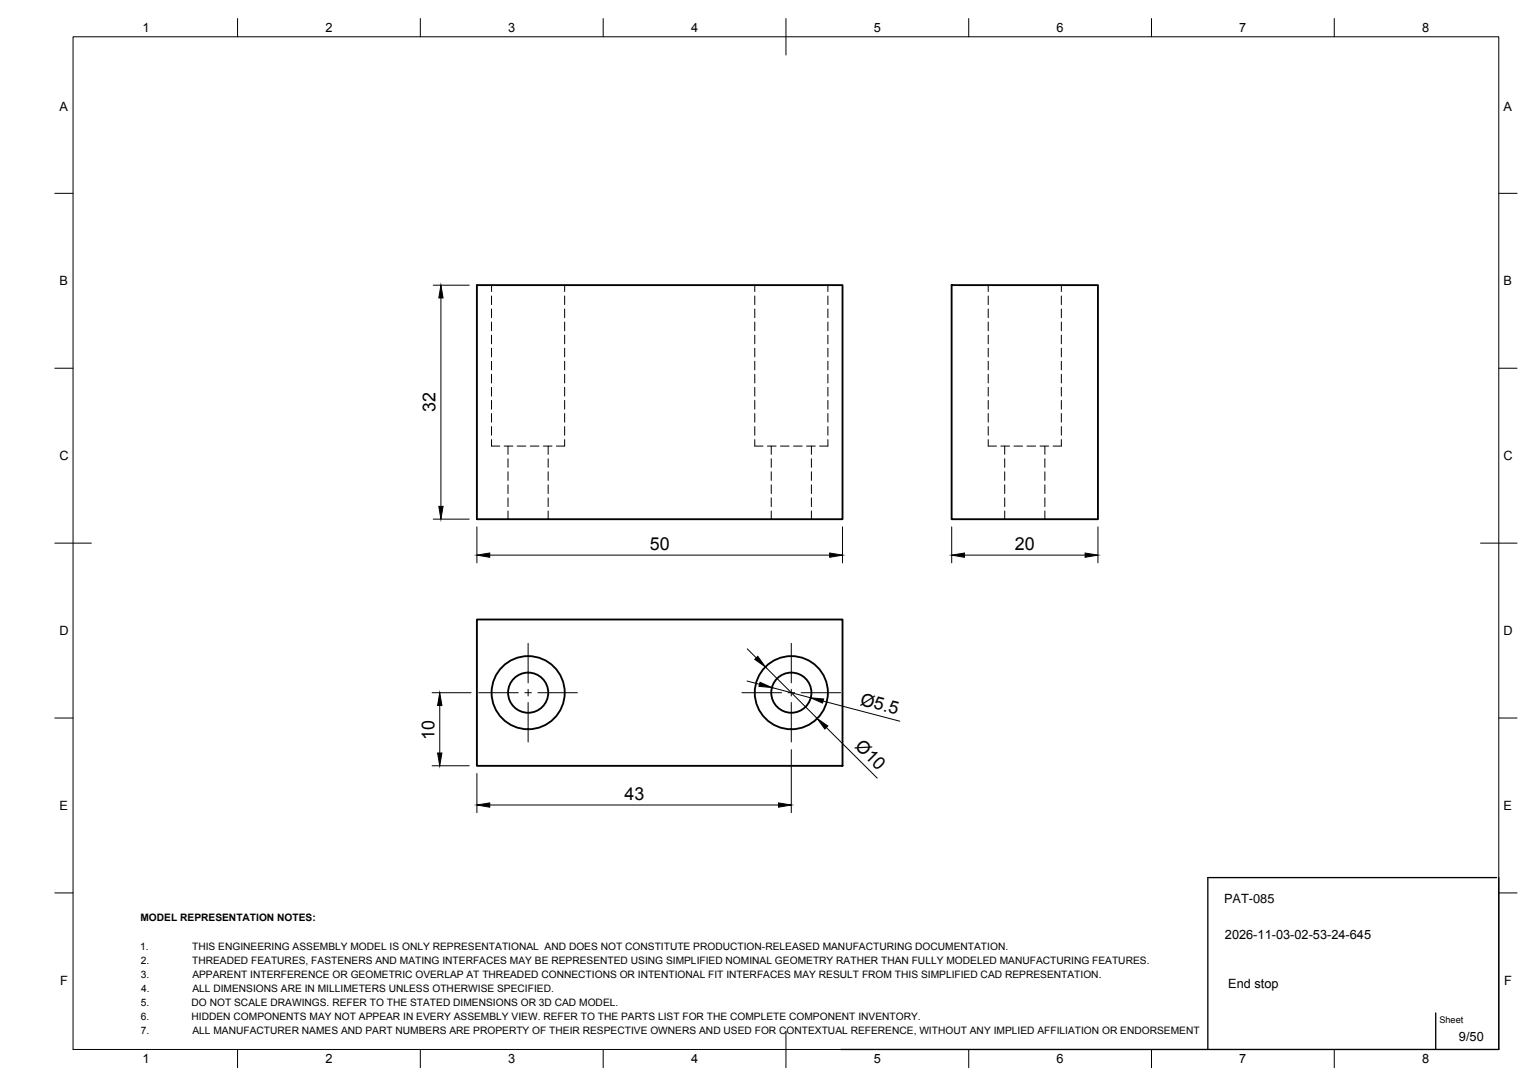
ISO-10303-21;
HEADER;
/* Generated by software containing ST-Developer
 * from STEP Tools, Inc. (www.steptools.com) 
 */

FILE_DESCRIPTION(
/* description */ ('Rack and pinion manual slide'),
/* implementation_level */ '2;1');

FILE_NAME(
/* name */ 'End stop.step',
/* time_stamp */ '2026-10-28T03:22:49-07:00',
/* author */ (''),
/* organization */ (''),
/* preprocessor_version */ 'ST-DEVELOPER v20.2',
/* originating_system */ 'Autodesk Translation Framework v15.17.0.0',
/* authorisation */ '');

FILE_SCHEMA (('AUTOMOTIVE_DESIGN { 1 0 10303 214 3 1 1 }'));
ENDSEC;

DATA;
#10=MECHANICAL_DESIGN_GEOMETRIC_PRESENTATION_REPRESENTATION('',(#736),#34851);
#644=SHAPE_REPRESENTATION_RELATIONSHIP('SRR','None',#35079,#690);
#690=ADVANCED_BREP_SHAPE_REPRESENTATION('',(#789),#34804);
#736=STYLED_ITEM('',(#35404),#789);
#789=MANIFOLD_SOLID_BREP('Body1',#13756);
#873=FACE_BOUND('',#2360,.T.);
#874=FACE_BOUND('',#2363,.T.);
#875=FACE_BOUND('',#2371,.T.);
#876=FACE_BOUND('',#2372,.T.);
#877=FACE_BOUND('',#2374,.T.);
#878=FACE_BOUND('',#2375,.T.);
#1068=PLANE('',#14411);
#1069=PLANE('',#14416);
#1070=PLANE('',#14422);
#1071=PLANE('',#14423);
#1072=PLANE('',#14424);
#1073=PLANE('',#14425);
#1074=PLANE('',#14426);
#1075=PLANE('',#14427);
#1579=FACE_OUTER_BOUND('',#2358,.T.);
#1580=FACE_OUTER_BOUND('',#2359,.T.);
#1581=FACE_OUTER_BOUND('',#2361,.T.);
#1582=FACE_OUTER_BOUND('',#2362,.T.);
#1583=FACE_OUTER_BOUND('',#2364,.T.);
#1584=FACE_OUTER_BOUND('',#2365,.T.);
#1585=FACE_OUTER_BOUND('',#2366,.T.);
#1586=FACE_OUTER_BOUND('',#2367,.T.);
#1587=FACE_OUTER_BOUND('',#2368,.T.);
#1588=FACE_OUTER_BOUND('',#2369,.T.);
#1589=FACE_OUTER_BOUND('',#2370,.T.);
#1590=FACE_OUTER_BOUND('',#2373,.T.);
#2358=EDGE_LOOP('',(#9450,#9451,#9452,#9453));
#2359=EDGE_LOOP('',(#9454));
#2360=EDGE_LOOP('',(#9455));
#2361=EDGE_LOOP('',(#9456,#9457,#9458,#9459));
#2362=EDGE_LOOP('',(#9460));
#2363=EDGE_LOOP('',(#9461));
#2364=EDGE_LOOP('',(#9462,#9463,#9464,#9465));
#2365=EDGE_LOOP('',(#9466,#9467,#9468,#9469));
#2366=EDGE_LOOP('',(#9470,#9471,#9472,#9473));
#2367=EDGE_LOOP('',(#9474,#9475,#9476,#9477));
#2368=EDGE_LOOP('',(#9478,#9479,#9480,#9481));
#2369=EDGE_LOOP('',(#9482,#9483,#9484,#9485));
#2370=EDGE_LOOP('',(#9486,#9487,#9488,#9489));
#2371=EDGE_LOOP('',(#9490));
#2372=EDGE_LOOP('',(#9491));
#2373=EDGE_LOOP('',(#9492,#9493,#9494,#9495));
#2374=EDGE_LOOP('',(#9496));
#2375=EDGE_LOOP('',(#9497));
#3292=LINE('',#19692,#4583);
#3293=LINE('',#19701,#4584);
#3294=LINE('',#19709,#4585);
#3295=LINE('',#19713,#4586);
#3296=LINE('',#19717,#4587);
#3297=LINE('',#19719,#4588);
#3298=LINE('',#19721,#4589);
#3299=LINE('',#19722,#4590);
#3300=LINE('',#19725,#4591);
#3301=LINE('',#19727,#4592);
#3302=LINE('',#19728,#4593);
#3303=LINE('',#19731,#4594);
#3304=LINE('',#19733,#4595);
#3305=LINE('',#19734,#4596);
#3306=LINE('',#19736,#4597);
#3307=LINE('',#19737,#4598);
#4583=VECTOR('',#15854,0.5);
#4584=VECTOR('',#15865,0.5);
#4585=VECTOR('',#15876,0.275);
#4586=VECTOR('',#15881,0.275);
#4587=VECTOR('',#15884,1.);
#4588=VECTOR('',#15885,1.);
#4589=VECTOR('',#15886,1.);
#4590=VECTOR('',#15887,1.);
#4591=VECTOR('',#15890,1.);
#4592=VECTOR('',#15891,1.);
#4593=VECTOR('',#15892,1.);
#4594=VECTOR('',#15895,1.);
#4595=VECTOR('',#15896,1.);
#4596=VECTOR('',#15897,1.);
#4597=VECTOR('',#15900,1.);
#4598=VECTOR('',#15901,1.);
#5846=CIRCLE('',#14409,0.5);
#5847=CIRCLE('',#14410,0.5);
#5848=CIRCLE('',#14412,0.275);
#5849=CIRCLE('',#14414,0.5);
#5850=CIRCLE('',#14415,0.5);
#5851=CIRCLE('',#14417,0.275);
#5852=CIRCLE('',#14419,0.275);
#5853=CIRCLE('',#14421,0.275);
#6296=VERTEX_POINT('',#19689);
#6297=VERTEX_POINT('',#19691);
#6298=VERTEX_POINT('',#19695);
#6299=VERTEX_POINT('',#19698);
#6300=VERTEX_POINT('',#19700);
#6301=VERTEX_POINT('',#19704);
#6302=VERTEX_POINT('',#19707);
#6303=VERTEX_POINT('',#19711);
#6304=VERTEX_POINT('',#19715);
#6305=VERTEX_POINT('',#19716);
#6306=VERTEX_POINT('',#19718);
#6307=VERTEX_POINT('',#19720);
#6308=VERTEX_POINT('',#19724);
#6309=VERTEX_POINT('',#19726);
#6310=VERTEX_POINT('',#19730);
#6311=VERTEX_POINT('',#19732);
#7537=EDGE_CURVE('',#6296,#6296,#5846,.T.);
#7538=EDGE_CURVE('',#6296,#6297,#3292,.T.);
#7539=EDGE_CURVE('',#6297,#6297,#5847,.T.);
#7540=EDGE_CURVE('',#6298,#6298,#5848,.T.);
#7541=EDGE_CURVE('',#6299,#6299,#5849,.T.);
#7542=EDGE_CURVE('',#6299,#6300,#3293,.T.);
#7543=EDGE_CURVE('',#6300,#6300,#5850,.T.);
#7544=EDGE_CURVE('',#6301,#6301,#5851,.T.);
#7545=EDGE_CURVE('',#6302,#6302,#5852,.T.);
#7546=EDGE_CURVE('',#6302,#6298,#3294,.T.);
#7547=EDGE_CURVE('',#6303,#6303,#5853,.T.);
#7548=EDGE_CURVE('',#6303,#6301,#3295,.T.);
#7549=EDGE_CURVE('',#6304,#6305,#3296,.T.);
#7550=EDGE_CURVE('',#6305,#6306,#3297,.T.);
#7551=EDGE_CURVE('',#6307,#6306,#3298,.T.);
#7552=EDGE_CURVE('',#6304,#6307,#3299,.T.);
#7553=EDGE_CURVE('',#6308,#6304,#3300,.T.);
#7554=EDGE_CURVE('',#6309,#6307,#3301,.T.);
#7555=EDGE_CURVE('',#6308,#6309,#3302,.T.);
#7556=EDGE_CURVE('',#6310,#6308,#3303,.T.);
#7557=EDGE_CURVE('',#6311,#6309,#3304,.T.);
#7558=EDGE_CURVE('',#6310,#6311,#3305,.T.);
#7559=EDGE_CURVE('',#6305,#6310,#3306,.T.);
#7560=EDGE_CURVE('',#6306,#6311,#3307,.T.);
#9450=ORIENTED_EDGE('',*,*,#7537,.F.);
#9451=ORIENTED_EDGE('',*,*,#7538,.T.);
#9452=ORIENTED_EDGE('',*,*,#7539,.F.);
#9453=ORIENTED_EDGE('',*,*,#7538,.F.);
#9454=ORIENTED_EDGE('',*,*,#7537,.T.);
#9455=ORIENTED_EDGE('',*,*,#7540,.F.);
#9456=ORIENTED_EDGE('',*,*,#7541,.F.);
#9457=ORIENTED_EDGE('',*,*,#7542,.T.);
#9458=ORIENTED_EDGE('',*,*,#7543,.F.);
#9459=ORIENTED_EDGE('',*,*,#7542,.F.);
#9460=ORIENTED_EDGE('',*,*,#7541,.T.);
#9461=ORIENTED_EDGE('',*,*,#7544,.F.);
#9462=ORIENTED_EDGE('',*,*,#7545,.F.);
#9463=ORIENTED_EDGE('',*,*,#7546,.T.);
#9464=ORIENTED_EDGE('',*,*,#7540,.T.);
#9465=ORIENTED_EDGE('',*,*,#7546,.F.);
#9466=ORIENTED_EDGE('',*,*,#7547,.F.);
#9467=ORIENTED_EDGE('',*,*,#7548,.T.);
#9468=ORIENTED_EDGE('',*,*,#7544,.T.);
#9469=ORIENTED_EDGE('',*,*,#7548,.F.);
#9470=ORIENTED_EDGE('',*,*,#7549,.T.);
#9471=ORIENTED_EDGE('',*,*,#7550,.T.);
#9472=ORIENTED_EDGE('',*,*,#7551,.F.);
#9473=ORIENTED_EDGE('',*,*,#7552,.F.);
#9474=ORIENTED_EDGE('',*,*,#7553,.T.);
#9475=ORIENTED_EDGE('',*,*,#7552,.T.);
#9476=ORIENTED_EDGE('',*,*,#7554,.F.);
#9477=ORIENTED_EDGE('',*,*,#7555,.F.);
#9478=ORIENTED_EDGE('',*,*,#7556,.T.);
#9479=ORIENTED_EDGE('',*,*,#7555,.T.);
#9480=ORIENTED_EDGE('',*,*,#7557,.F.);
#9481=ORIENTED_EDGE('',*,*,#7558,.F.);
#9482=ORIENTED_EDGE('',*,*,#7559,.T.);
#9483=ORIENTED_EDGE('',*,*,#7558,.T.);
#9484=ORIENTED_EDGE('',*,*,#7560,.F.);
#9485=ORIENTED_EDGE('',*,*,#7550,.F.);
#9486=ORIENTED_EDGE('',*,*,#7560,.T.);
#9487=ORIENTED_EDGE('',*,*,#7557,.T.);
#9488=ORIENTED_EDGE('',*,*,#7554,.T.);
#9489=ORIENTED_EDGE('',*,*,#7551,.T.);
#9490=ORIENTED_EDGE('',*,*,#7539,.T.);
#9491=ORIENTED_EDGE('',*,*,#7543,.T.);
#9492=ORIENTED_EDGE('',*,*,#7559,.F.);
#9493=ORIENTED_EDGE('',*,*,#7549,.F.);
#9494=ORIENTED_EDGE('',*,*,#7553,.F.);
#9495=ORIENTED_EDGE('',*,*,#7556,.F.);
#9496=ORIENTED_EDGE('',*,*,#7545,.T.);
#9497=ORIENTED_EDGE('',*,*,#7547,.T.);
#12864=CYLINDRICAL_SURFACE('',#14408,0.5);
#12865=CYLINDRICAL_SURFACE('',#14413,0.5);
#12866=CYLINDRICAL_SURFACE('',#14418,0.275);
#12867=CYLINDRICAL_SURFACE('',#14420,0.275);
#13057=ADVANCED_FACE('',(#1579),#12864,.F.);
#13058=ADVANCED_FACE('',(#1580,#873),#1068,.T.);
#13059=ADVANCED_FACE('',(#1581),#12865,.F.);
#13060=ADVANCED_FACE('',(#1582,#874),#1069,.T.);
#13061=ADVANCED_FACE('',(#1583),#12866,.F.);
#13062=ADVANCED_FACE('',(#1584),#12867,.F.);
#13063=ADVANCED_FACE('',(#1585),#1070,.T.);
#13064=ADVANCED_FACE('',(#1586),#1071,.T.);
#13065=ADVANCED_FACE('',(#1587),#1072,.T.);
#13066=ADVANCED_FACE('',(#1588),#1073,.T.);
#13067=ADVANCED_FACE('',(#1589,#875,#876),#1074,.T.);
#13068=ADVANCED_FACE('',(#1590,#877,#878),#1075,.F.);
#13756=CLOSED_SHELL('',(#13057,#13058,#13059,#13060,#13061,#13062,#13063,
#13064,#13065,#13066,#13067,#13068));
#14407=AXIS2_PLACEMENT_3D('',#19687,#15848,#15849);
#14408=AXIS2_PLACEMENT_3D('',#19688,#15850,#15851);
#14409=AXIS2_PLACEMENT_3D('',#19690,#15852,#15853);
#14410=AXIS2_PLACEMENT_3D('',#19693,#15855,#15856);
#14411=AXIS2_PLACEMENT_3D('',#19694,#15857,#15858);
#14412=AXIS2_PLACEMENT_3D('',#19696,#15859,#15860);
#14413=AXIS2_PLACEMENT_3D('',#19697,#15861,#15862);
#14414=AXIS2_PLACEMENT_3D('',#19699,#15863,#15864);
#14415=AXIS2_PLACEMENT_3D('',#19702,#15866,#15867);
#14416=AXIS2_PLACEMENT_3D('',#19703,#15868,#15869);
#14417=AXIS2_PLACEMENT_3D('',#19705,#15870,#15871);
#14418=AXIS2_PLACEMENT_3D('',#19706,#15872,#15873);
#14419=AXIS2_PLACEMENT_3D('',#19708,#15874,#15875);
#14420=AXIS2_PLACEMENT_3D('',#19710,#15877,#15878);
#14421=AXIS2_PLACEMENT_3D('',#19712,#15879,#15880);
#14422=AXIS2_PLACEMENT_3D('',#19714,#15882,#15883);
#14423=AXIS2_PLACEMENT_3D('',#19723,#15888,#15889);
#14424=AXIS2_PLACEMENT_3D('',#19729,#15893,#15894);
#14425=AXIS2_PLACEMENT_3D('',#19735,#15898,#15899);
#14426=AXIS2_PLACEMENT_3D('',#19738,#15902,#15903);
#14427=AXIS2_PLACEMENT_3D('',#19739,#15904,#15905);
#15848=DIRECTION('axis',(0.,0.,1.));
#15849=DIRECTION('refdir',(1.,0.,0.));
#15850=DIRECTION('center_axis',(0.,0.,1.));
#15851=DIRECTION('ref_axis',(1.,0.,0.));
#15852=DIRECTION('center_axis',(0.,0.,1.));
#15853=DIRECTION('ref_axis',(1.,0.,0.));
#15854=DIRECTION('',(0.,0.,1.));
#15855=DIRECTION('center_axis',(0.,0.,-1.));
#15856=DIRECTION('ref_axis',(1.,0.,0.));
#15857=DIRECTION('center_axis',(0.,0.,1.));
#15858=DIRECTION('ref_axis',(1.,0.,0.));
#15859=DIRECTION('center_axis',(0.,0.,1.));
#15860=DIRECTION('ref_axis',(1.,0.,0.));
#15861=DIRECTION('center_axis',(0.,0.,1.));
#15862=DIRECTION('ref_axis',(1.,0.,0.));
#15863=DIRECTION('center_axis',(0.,0.,1.));
#15864=DIRECTION('ref_axis',(1.,0.,0.));
#15865=DIRECTION('',(0.,0.,1.));
#15866=DIRECTION('center_axis',(0.,0.,-1.));
#15867=DIRECTION('ref_axis',(1.,0.,0.));
#15868=DIRECTION('center_axis',(0.,0.,1.));
#15869=DIRECTION('ref_axis',(1.,0.,0.));
#15870=DIRECTION('center_axis',(0.,0.,1.));
#15871=DIRECTION('ref_axis',(1.,0.,0.));
#15872=DIRECTION('center_axis',(0.,0.,1.));
#15873=DIRECTION('ref_axis',(1.,0.,0.));
#15874=DIRECTION('center_axis',(0.,0.,1.));
#15875=DIRECTION('ref_axis',(1.,0.,0.));
#15876=DIRECTION('',(0.,0.,1.));
#15877=DIRECTION('center_axis',(0.,0.,1.));
#15878=DIRECTION('ref_axis',(1.,0.,0.));
#15879=DIRECTION('center_axis',(0.,0.,1.));
#15880=DIRECTION('ref_axis',(1.,0.,0.));
#15881=DIRECTION('',(0.,0.,1.));
#15882=DIRECTION('center_axis',(0.,1.,0.));
#15883=DIRECTION('ref_axis',(-1.,0.,0.));
#15884=DIRECTION('',(-1.,0.,0.));
#15885=DIRECTION('',(0.,0.,1.));
#15886=DIRECTION('',(-1.,0.,0.));
#15887=DIRECTION('',(0.,0.,1.));
#15888=DIRECTION('center_axis',(1.,0.,0.));
#15889=DIRECTION('ref_axis',(0.,1.,0.));
#15890=DIRECTION('',(0.,1.,0.));
#15891=DIRECTION('',(0.,1.,0.));
#15892=DIRECTION('',(0.,0.,1.));
#15893=DIRECTION('center_axis',(0.,-1.,0.));
#15894=DIRECTION('ref_axis',(1.,0.,0.));
#15895=DIRECTION('',(1.,0.,0.));
#15896=DIRECTION('',(1.,0.,0.));
#15897=DIRECTION('',(0.,0.,1.));
#15898=DIRECTION('center_axis',(-1.,0.,0.));
#15899=DIRECTION('ref_axis',(0.,-1.,0.));
#15900=DIRECTION('',(0.,-1.,0.));
#15901=DIRECTION('',(0.,-1.,0.));
#15902=DIRECTION('center_axis',(0.,0.,1.));
#15903=DIRECTION('ref_axis',(1.,0.,0.));
#15904=DIRECTION('center_axis',(0.,0.,1.));
#15905=DIRECTION('ref_axis',(1.,0.,0.));
#19687=CARTESIAN_POINT('',(0.,0.,0.));
#19688=CARTESIAN_POINT('Origin',(-4.2,-1.8,4.8));
#19689=CARTESIAN_POINT('',(-4.7,-1.8,4.8));
#19690=CARTESIAN_POINT('Origin',(-4.2,-1.8,4.8));
#19691=CARTESIAN_POINT('',(-4.7,-1.8,7.));
#19692=CARTESIAN_POINT('',(-4.7,-1.8,4.8));
#19693=CARTESIAN_POINT('Origin',(-4.2,-1.8,7.));
#19694=CARTESIAN_POINT('Origin',(-4.2,-1.8,4.8));
#19695=CARTESIAN_POINT('',(-4.475,-1.8,4.8));
#19696=CARTESIAN_POINT('Origin',(-4.2,-1.8,4.8));
#19697=CARTESIAN_POINT('Origin',(-4.2,1.8,4.8));
#19698=CARTESIAN_POINT('',(-4.7,1.8,4.8));
#19699=CARTESIAN_POINT('Origin',(-4.2,1.8,4.8));
#19700=CARTESIAN_POINT('',(-4.7,1.8,7.));
#19701=CARTESIAN_POINT('',(-4.7,1.8,4.8));
#19702=CARTESIAN_POINT('Origin',(-4.2,1.8,7.));
#19703=CARTESIAN_POINT('Origin',(-4.2,1.8,4.8));
#19704=CARTESIAN_POINT('',(-4.475,1.8,4.8));
#19705=CARTESIAN_POINT('Origin',(-4.2,1.8,4.8));
#19706=CARTESIAN_POINT('Origin',(-4.2,-1.8,3.7));
#19707=CARTESIAN_POINT('',(-4.475,-1.8,3.8));
#19708=CARTESIAN_POINT('Origin',(-4.2,-1.8,3.8));
#19709=CARTESIAN_POINT('',(-4.475,-1.8,3.7));
#19710=CARTESIAN_POINT('Origin',(-4.2,1.8,3.7));
#19711=CARTESIAN_POINT('',(-4.475,1.8,3.8));
#19712=CARTESIAN_POINT('Origin',(-4.2,1.8,3.8));
#19713=CARTESIAN_POINT('',(-4.475,1.8,3.7));
#19714=CARTESIAN_POINT('Origin',(-3.2,2.5,3.8));
#19715=CARTESIAN_POINT('',(-3.2,2.5,3.8));
#19716=CARTESIAN_POINT('',(-5.2,2.5,3.8));
#19717=CARTESIAN_POINT('',(-3.2,2.5,3.8));
#19718=CARTESIAN_POINT('',(-5.2,2.5,7.));
#19719=CARTESIAN_POINT('',(-5.2,2.5,3.8));
#19720=CARTESIAN_POINT('',(-3.2,2.5,7.));
#19721=CARTESIAN_POINT('',(-3.2,2.5,7.));
#19722=CARTESIAN_POINT('',(-3.2,2.5,3.8));
#19723=CARTESIAN_POINT('Origin',(-3.2,-2.5,3.8));
#19724=CARTESIAN_POINT('',(-3.2,-2.5,3.8));
#19725=CARTESIAN_POINT('',(-3.2,-2.5,3.8));
#19726=CARTESIAN_POINT('',(-3.2,-2.5,7.));
#19727=CARTESIAN_POINT('',(-3.2,-2.5,7.));
#19728=CARTESIAN_POINT('',(-3.2,-2.5,3.8));
#19729=CARTESIAN_POINT('Origin',(-5.2,-2.5,3.8));
#19730=CARTESIAN_POINT('',(-5.2,-2.5,3.8));
#19731=CARTESIAN_POINT('',(-5.2,-2.5,3.8));
#19732=CARTESIAN_POINT('',(-5.2,-2.5,7.));
#19733=CARTESIAN_POINT('',(-5.2,-2.5,7.));
#19734=CARTESIAN_POINT('',(-5.2,-2.5,3.8));
#19735=CARTESIAN_POINT('Origin',(-5.2,2.5,3.8));
#19736=CARTESIAN_POINT('',(-5.2,2.5,3.8));
#19737=CARTESIAN_POINT('',(-5.2,2.5,7.));
#19738=CARTESIAN_POINT('Origin',(-4.2,0.,7.));
#19739=CARTESIAN_POINT('Origin',(-4.2,0.,3.8));
#34750=UNCERTAINTY_MEASURE_WITH_UNIT(LENGTH_MEASURE(0.001),#34852,
'DISTANCE_ACCURACY_VALUE',
'Maximum model space distance between geometric entities at asserted c
onnectivities');
#34797=UNCERTAINTY_MEASURE_WITH_UNIT(LENGTH_MEASURE(0.001),#34852,
'DISTANCE_ACCURACY_VALUE',
'Maximum model space distance between geometric entities at asserted c
onnectivities');
#34804=(
GEOMETRIC_REPRESENTATION_CONTEXT(3)
GLOBAL_UNCERTAINTY_ASSIGNED_CONTEXT((#34750))
GLOBAL_UNIT_ASSIGNED_CONTEXT((#34852,#34854,#34855))
REPRESENTATION_CONTEXT('','3D')
);
#34851=(
GEOMETRIC_REPRESENTATION_CONTEXT(3)
GLOBAL_UNCERTAINTY_ASSIGNED_CONTEXT((#34797))
GLOBAL_UNIT_ASSIGNED_CONTEXT((#34852,#34854,#34855))
REPRESENTATION_CONTEXT('','3D')
);
#34852=(
LENGTH_UNIT()
NAMED_UNIT(*)
SI_UNIT(.CENTI.,.METRE.)
);
#34854=(
NAMED_UNIT(*)
PLANE_ANGLE_UNIT()
SI_UNIT($,.RADIAN.)
);
#34855=(
NAMED_UNIT(*)
SI_UNIT($,.STERADIAN.)
SOLID_ANGLE_UNIT()
);
#34862=SHAPE_DEFINITION_REPRESENTATION(#34915,#35079);
#34915=PRODUCT_DEFINITION_SHAPE('',$,#35133);
#35079=SHAPE_REPRESENTATION('',(#14407),#34804);
#35126=PRODUCT_DEFINITION_CONTEXT('part definition',#35287,'design');
#35133=PRODUCT_DEFINITION('End stop','End stop',#35186,#35126);
#35186=PRODUCT_DEFINITION_FORMATION('',$,#35295);
#35287=APPLICATION_CONTEXT(
'Core Data for Automotive Mechanical Design Process');
#35288=PRODUCT_CONTEXT('part definition',#35287,'mechanical');
#35295=PRODUCT('End stop','End stop','End stop',(#35288));
#35398=COLOUR_RGB('Sky Blue',0.24,0.69,0.87);
#35399=FILL_AREA_STYLE_COLOUR('',#35398);
#35400=FILL_AREA_STYLE('',(#35399));
#35401=SURFACE_STYLE_FILL_AREA(#35400);
#35402=SURFACE_SIDE_STYLE('',(#35401));
#35403=SURFACE_STYLE_USAGE(.BOTH.,#35402);
#35404=PRESENTATION_STYLE_ASSIGNMENT((#35403));
ENDSEC;
END-ISO-10303-21;
